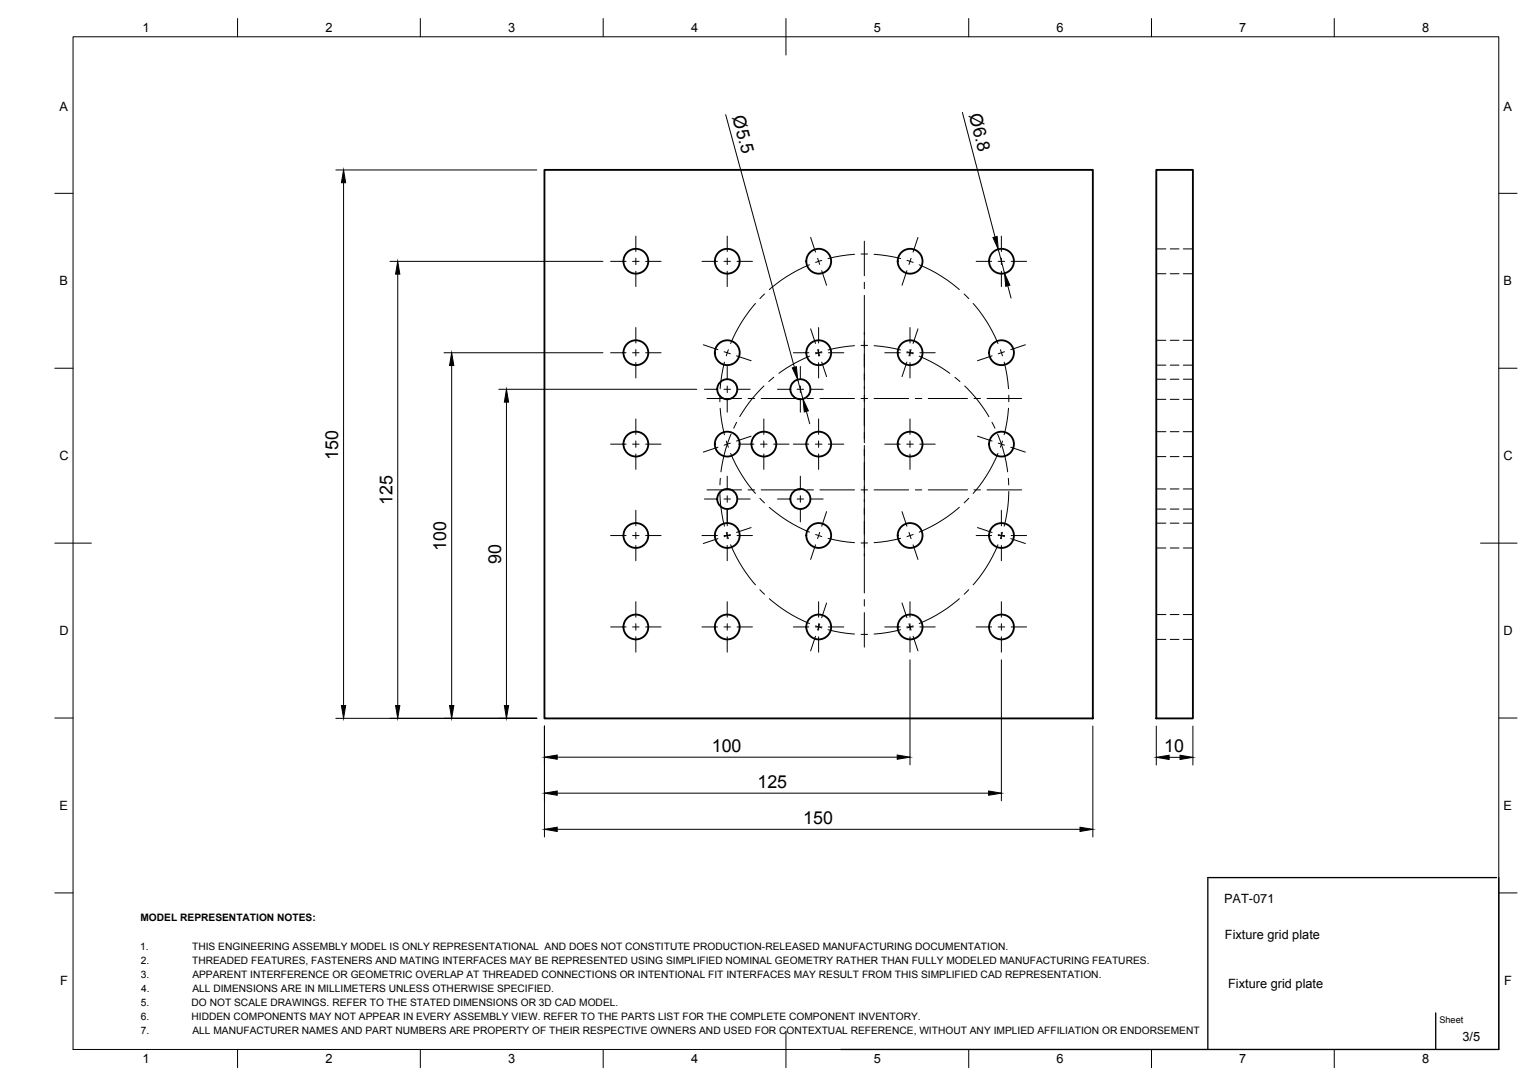
ISO-10303-21;
HEADER;
/* Generated by software containing ST-Developer
 * from STEP Tools, Inc. (www.steptools.com) 
 */

FILE_DESCRIPTION(
/* description */ ('Low-profile wedge edge clamp'),
/* implementation_level */ '2;1');

FILE_NAME(
/* name */ 'Fixture grid plate.step',
/* time_stamp */ '2026-10-29T15:58:13-07:00',
/* author */ (''),
/* organization */ (''),
/* preprocessor_version */ 'ST-DEVELOPER v20.2',
/* originating_system */ 'Autodesk Translation Framework v15.17.0.0',
/* authorisation */ '');

FILE_SCHEMA (('AUTOMOTIVE_DESIGN { 1 0 10303 214 3 1 1 }'));
ENDSEC;

DATA;
#10=MECHANICAL_DESIGN_GEOMETRIC_PRESENTATION_REPRESENTATION('',(#79),#2996);
#67=SHAPE_REPRESENTATION_RELATIONSHIP('SRR','None',#3029,#73);
#73=ADVANCED_BREP_SHAPE_REPRESENTATION('',(#85),#2990);
#79=STYLED_ITEM('',(#3140),#85);
#85=MANIFOLD_SOLID_BREP('Body1',#1708);
#90=FACE_BOUND('',#336,.T.);
#91=FACE_BOUND('',#337,.T.);
#92=FACE_BOUND('',#338,.T.);
#93=FACE_BOUND('',#339,.T.);
#94=FACE_BOUND('',#340,.T.);
#95=FACE_BOUND('',#341,.T.);
#96=FACE_BOUND('',#342,.T.);
#97=FACE_BOUND('',#343,.T.);
#98=FACE_BOUND('',#344,.T.);
#99=FACE_BOUND('',#345,.T.);
#100=FACE_BOUND('',#346,.T.);
#101=FACE_BOUND('',#347,.T.);
#102=FACE_BOUND('',#348,.T.);
#103=FACE_BOUND('',#349,.T.);
#104=FACE_BOUND('',#350,.T.);
#105=FACE_BOUND('',#351,.T.);
#106=FACE_BOUND('',#352,.T.);
#107=FACE_BOUND('',#353,.T.);
#108=FACE_BOUND('',#354,.T.);
#109=FACE_BOUND('',#355,.T.);
#110=FACE_BOUND('',#356,.T.);
#111=FACE_BOUND('',#357,.T.);
#112=FACE_BOUND('',#358,.T.);
#113=FACE_BOUND('',#359,.T.);
#114=FACE_BOUND('',#360,.T.);
#115=FACE_BOUND('',#361,.T.);
#116=FACE_BOUND('',#362,.T.);
#117=FACE_BOUND('',#363,.T.);
#118=FACE_BOUND('',#364,.T.);
#119=FACE_BOUND('',#365,.T.);
#120=FACE_BOUND('',#367,.T.);
#121=FACE_BOUND('',#368,.T.);
#122=FACE_BOUND('',#369,.T.);
#123=FACE_BOUND('',#370,.T.);
#124=FACE_BOUND('',#371,.T.);
#125=FACE_BOUND('',#372,.T.);
#126=FACE_BOUND('',#373,.T.);
#127=FACE_BOUND('',#374,.T.);
#128=FACE_BOUND('',#375,.T.);
#129=FACE_BOUND('',#376,.T.);
#130=FACE_BOUND('',#377,.T.);
#131=FACE_BOUND('',#378,.T.);
#132=FACE_BOUND('',#379,.T.);
#133=FACE_BOUND('',#380,.T.);
#134=FACE_BOUND('',#381,.T.);
#135=FACE_BOUND('',#382,.T.);
#136=FACE_BOUND('',#383,.T.);
#137=FACE_BOUND('',#384,.T.);
#138=FACE_BOUND('',#385,.T.);
#139=FACE_BOUND('',#386,.T.);
#140=FACE_BOUND('',#387,.T.);
#141=FACE_BOUND('',#388,.T.);
#142=FACE_BOUND('',#389,.T.);
#143=FACE_BOUND('',#390,.T.);
#144=FACE_BOUND('',#391,.T.);
#145=FACE_BOUND('',#392,.T.);
#146=FACE_BOUND('',#393,.T.);
#147=FACE_BOUND('',#394,.T.);
#148=FACE_BOUND('',#395,.T.);
#149=FACE_BOUND('',#396,.T.);
#162=PLANE('',#1875);
#163=PLANE('',#1876);
#164=PLANE('',#1877);
#165=PLANE('',#1878);
#166=PLANE('',#1879);
#167=PLANE('',#1880);
#208=FACE_OUTER_BOUND('',#301,.T.);
#209=FACE_OUTER_BOUND('',#302,.T.);
#210=FACE_OUTER_BOUND('',#303,.T.);
#211=FACE_OUTER_BOUND('',#304,.T.);
#212=FACE_OUTER_BOUND('',#305,.T.);
#213=FACE_OUTER_BOUND('',#306,.T.);
#214=FACE_OUTER_BOUND('',#307,.T.);
#215=FACE_OUTER_BOUND('',#308,.T.);
#216=FACE_OUTER_BOUND('',#309,.T.);
#217=FACE_OUTER_BOUND('',#310,.T.);
#218=FACE_OUTER_BOUND('',#311,.T.);
#219=FACE_OUTER_BOUND('',#312,.T.);
#220=FACE_OUTER_BOUND('',#313,.T.);
#221=FACE_OUTER_BOUND('',#314,.T.);
#222=FACE_OUTER_BOUND('',#315,.T.);
#223=FACE_OUTER_BOUND('',#316,.T.);
#224=FACE_OUTER_BOUND('',#317,.T.);
#225=FACE_OUTER_BOUND('',#318,.T.);
#226=FACE_OUTER_BOUND('',#319,.T.);
#227=FACE_OUTER_BOUND('',#320,.T.);
#228=FACE_OUTER_BOUND('',#321,.T.);
#229=FACE_OUTER_BOUND('',#322,.T.);
#230=FACE_OUTER_BOUND('',#323,.T.);
#231=FACE_OUTER_BOUND('',#324,.T.);
#232=FACE_OUTER_BOUND('',#325,.T.);
#233=FACE_OUTER_BOUND('',#326,.T.);
#234=FACE_OUTER_BOUND('',#327,.T.);
#235=FACE_OUTER_BOUND('',#328,.T.);
#236=FACE_OUTER_BOUND('',#329,.T.);
#237=FACE_OUTER_BOUND('',#330,.T.);
#238=FACE_OUTER_BOUND('',#331,.T.);
#239=FACE_OUTER_BOUND('',#332,.T.);
#240=FACE_OUTER_BOUND('',#333,.T.);
#241=FACE_OUTER_BOUND('',#334,.T.);
#242=FACE_OUTER_BOUND('',#335,.T.);
#243=FACE_OUTER_BOUND('',#366,.T.);
#301=EDGE_LOOP('',(#1145,#1146,#1147,#1148));
#302=EDGE_LOOP('',(#1149,#1150,#1151,#1152));
#303=EDGE_LOOP('',(#1153,#1154,#1155,#1156));
#304=EDGE_LOOP('',(#1157,#1158,#1159,#1160));
#305=EDGE_LOOP('',(#1161,#1162,#1163,#1164));
#306=EDGE_LOOP('',(#1165,#1166,#1167,#1168));
#307=EDGE_LOOP('',(#1169,#1170,#1171,#1172));
#308=EDGE_LOOP('',(#1173,#1174,#1175,#1176));
#309=EDGE_LOOP('',(#1177,#1178,#1179,#1180));
#310=EDGE_LOOP('',(#1181,#1182,#1183,#1184));
#311=EDGE_LOOP('',(#1185,#1186,#1187,#1188));
#312=EDGE_LOOP('',(#1189,#1190,#1191,#1192));
#313=EDGE_LOOP('',(#1193,#1194,#1195,#1196));
#314=EDGE_LOOP('',(#1197,#1198,#1199,#1200));
#315=EDGE_LOOP('',(#1201,#1202,#1203,#1204));
#316=EDGE_LOOP('',(#1205,#1206,#1207,#1208));
#317=EDGE_LOOP('',(#1209,#1210,#1211,#1212));
#318=EDGE_LOOP('',(#1213,#1214,#1215,#1216));
#319=EDGE_LOOP('',(#1217,#1218,#1219,#1220));
#320=EDGE_LOOP('',(#1221,#1222,#1223,#1224));
#321=EDGE_LOOP('',(#1225,#1226,#1227,#1228));
#322=EDGE_LOOP('',(#1229,#1230,#1231,#1232));
#323=EDGE_LOOP('',(#1233,#1234,#1235,#1236));
#324=EDGE_LOOP('',(#1237,#1238,#1239,#1240));
#325=EDGE_LOOP('',(#1241,#1242,#1243,#1244));
#326=EDGE_LOOP('',(#1245,#1246,#1247,#1248));
#327=EDGE_LOOP('',(#1249,#1250,#1251,#1252));
#328=EDGE_LOOP('',(#1253,#1254,#1255,#1256));
#329=EDGE_LOOP('',(#1257,#1258,#1259,#1260));
#330=EDGE_LOOP('',(#1261,#1262,#1263,#1264));
#331=EDGE_LOOP('',(#1265,#1266,#1267,#1268));
#332=EDGE_LOOP('',(#1269,#1270,#1271,#1272));
#333=EDGE_LOOP('',(#1273,#1274,#1275,#1276));
#334=EDGE_LOOP('',(#1277,#1278,#1279,#1280));
#335=EDGE_LOOP('',(#1281,#1282,#1283,#1284));
#336=EDGE_LOOP('',(#1285));
#337=EDGE_LOOP('',(#1286));
#338=EDGE_LOOP('',(#1287));
#339=EDGE_LOOP('',(#1288));
#340=EDGE_LOOP('',(#1289));
#341=EDGE_LOOP('',(#1290));
#342=EDGE_LOOP('',(#1291));
#343=EDGE_LOOP('',(#1292));
#344=EDGE_LOOP('',(#1293));
#345=EDGE_LOOP('',(#1294));
#346=EDGE_LOOP('',(#1295));
#347=EDGE_LOOP('',(#1296));
#348=EDGE_LOOP('',(#1297));
#349=EDGE_LOOP('',(#1298));
#350=EDGE_LOOP('',(#1299));
#351=EDGE_LOOP('',(#1300));
#352=EDGE_LOOP('',(#1301));
#353=EDGE_LOOP('',(#1302));
#354=EDGE_LOOP('',(#1303));
#355=EDGE_LOOP('',(#1304));
#356=EDGE_LOOP('',(#1305));
#357=EDGE_LOOP('',(#1306));
#358=EDGE_LOOP('',(#1307));
#359=EDGE_LOOP('',(#1308));
#360=EDGE_LOOP('',(#1309));
#361=EDGE_LOOP('',(#1310));
#362=EDGE_LOOP('',(#1311));
#363=EDGE_LOOP('',(#1312));
#364=EDGE_LOOP('',(#1313));
#365=EDGE_LOOP('',(#1314));
#366=EDGE_LOOP('',(#1315,#1316,#1317,#1318));
#367=EDGE_LOOP('',(#1319));
#368=EDGE_LOOP('',(#1320));
#369=EDGE_LOOP('',(#1321));
#370=EDGE_LOOP('',(#1322));
#371=EDGE_LOOP('',(#1323));
#372=EDGE_LOOP('',(#1324));
#373=EDGE_LOOP('',(#1325));
#374=EDGE_LOOP('',(#1326));
#375=EDGE_LOOP('',(#1327));
#376=EDGE_LOOP('',(#1328));
#377=EDGE_LOOP('',(#1329));
#378=EDGE_LOOP('',(#1330));
#379=EDGE_LOOP('',(#1331));
#380=EDGE_LOOP('',(#1332));
#381=EDGE_LOOP('',(#1333));
#382=EDGE_LOOP('',(#1334));
#383=EDGE_LOOP('',(#1335));
#384=EDGE_LOOP('',(#1336));
#385=EDGE_LOOP('',(#1337));
#386=EDGE_LOOP('',(#1338));
#387=EDGE_LOOP('',(#1339));
#388=EDGE_LOOP('',(#1340));
#389=EDGE_LOOP('',(#1341));
#390=EDGE_LOOP('',(#1342));
#391=EDGE_LOOP('',(#1343));
#392=EDGE_LOOP('',(#1344));
#393=EDGE_LOOP('',(#1345));
#394=EDGE_LOOP('',(#1346));
#395=EDGE_LOOP('',(#1347));
#396=EDGE_LOOP('',(#1348));
#466=LINE('',#2508,#585);
#467=LINE('',#2514,#586);
#468=LINE('',#2520,#587);
#469=LINE('',#2526,#588);
#470=LINE('',#2532,#589);
#471=LINE('',#2538,#590);
#472=LINE('',#2544,#591);
#473=LINE('',#2550,#592);
#474=LINE('',#2556,#593);
#475=LINE('',#2562,#594);
#476=LINE('',#2568,#595);
#477=LINE('',#2574,#596);
#478=LINE('',#2580,#597);
#479=LINE('',#2586,#598);
#480=LINE('',#2592,#599);
#481=LINE('',#2598,#600);
#482=LINE('',#2604,#601);
#483=LINE('',#2610,#602);
#484=LINE('',#2616,#603);
#485=LINE('',#2622,#604);
#486=LINE('',#2628,#605);
#487=LINE('',#2634,#606);
#488=LINE('',#2640,#607);
#489=LINE('',#2646,#608);
#490=LINE('',#2652,#609);
#491=LINE('',#2658,#610);
#492=LINE('',#2664,#611);
#493=LINE('',#2670,#612);
#494=LINE('',#2676,#613);
#495=LINE('',#2682,#614);
#496=LINE('',#2687,#615);
#497=LINE('',#2689,#616);
#498=LINE('',#2691,#617);
#499=LINE('',#2692,#618);
#500=LINE('',#2695,#619);
#501=LINE('',#2697,#620);
#502=LINE('',#2698,#621);
#503=LINE('',#2701,#622);
#504=LINE('',#2703,#623);
#505=LINE('',#2704,#624);
#506=LINE('',#2706,#625);
#507=LINE('',#2707,#626);
#585=VECTOR('',#1992,0.275);
#586=VECTOR('',#1999,0.275);
#587=VECTOR('',#2006,0.275);
#588=VECTOR('',#2013,0.275);
#589=VECTOR('',#2020,0.34);
#590=VECTOR('',#2027,0.34);
#591=VECTOR('',#2034,0.34);
#592=VECTOR('',#2041,0.34);
#593=VECTOR('',#2048,0.34);
#594=VECTOR('',#2055,0.34);
#595=VECTOR('',#2062,0.34);
#596=VECTOR('',#2069,0.34);
#597=VECTOR('',#2076,0.34);
#598=VECTOR('',#2083,0.34);
#599=VECTOR('',#2090,0.34);
#600=VECTOR('',#2097,0.34);
#601=VECTOR('',#2104,0.34);
#602=VECTOR('',#2111,0.34);
#603=VECTOR('',#2118,0.34);
#604=VECTOR('',#2125,0.34);
#605=VECTOR('',#2132,0.34);
#606=VECTOR('',#2139,0.34);
#607=VECTOR('',#2146,0.34);
#608=VECTOR('',#2153,0.34);
#609=VECTOR('',#2160,0.34);
#610=VECTOR('',#2167,0.34);
#611=VECTOR('',#2174,0.34);
#612=VECTOR('',#2181,0.34);
#613=VECTOR('',#2188,0.34);
#614=VECTOR('',#2195,0.34);
#615=VECTOR('',#2200,1.);
#616=VECTOR('',#2201,1.);
#617=VECTOR('',#2202,1.);
#618=VECTOR('',#2203,1.);
#619=VECTOR('',#2206,1.);
#620=VECTOR('',#2207,1.);
#621=VECTOR('',#2208,1.);
#622=VECTOR('',#2211,1.);
#623=VECTOR('',#2212,1.);
#624=VECTOR('',#2213,1.);
#625=VECTOR('',#2216,1.);
#626=VECTOR('',#2217,1.);
#704=CIRCLE('',#1786,0.275);
#705=CIRCLE('',#1787,0.275);
#706=CIRCLE('',#1789,0.275);
#707=CIRCLE('',#1790,0.275);
#708=CIRCLE('',#1792,0.275);
#709=CIRCLE('',#1793,0.275);
#710=CIRCLE('',#1795,0.275);
#711=CIRCLE('',#1796,0.275);
#712=CIRCLE('',#1798,0.34);
#713=CIRCLE('',#1799,0.34);
#714=CIRCLE('',#1801,0.34);
#715=CIRCLE('',#1802,0.34);
#716=CIRCLE('',#1804,0.34);
#717=CIRCLE('',#1805,0.34);
#718=CIRCLE('',#1807,0.34);
#719=CIRCLE('',#1808,0.34);
#720=CIRCLE('',#1810,0.34);
#721=CIRCLE('',#1811,0.34);
#722=CIRCLE('',#1813,0.34);
#723=CIRCLE('',#1814,0.34);
#724=CIRCLE('',#1816,0.34);
#725=CIRCLE('',#1817,0.34);
#726=CIRCLE('',#1819,0.34);
#727=CIRCLE('',#1820,0.34);
#728=CIRCLE('',#1822,0.34);
#729=CIRCLE('',#1823,0.34);
#730=CIRCLE('',#1825,0.34);
#731=CIRCLE('',#1826,0.34);
#732=CIRCLE('',#1828,0.34);
#733=CIRCLE('',#1829,0.34);
#734=CIRCLE('',#1831,0.34);
#735=CIRCLE('',#1832,0.34);
#736=CIRCLE('',#1834,0.34);
#737=CIRCLE('',#1835,0.34);
#738=CIRCLE('',#1837,0.34);
#739=CIRCLE('',#1838,0.34);
#740=CIRCLE('',#1840,0.34);
#741=CIRCLE('',#1841,0.34);
#742=CIRCLE('',#1843,0.34);
#743=CIRCLE('',#1844,0.34);
#744=CIRCLE('',#1846,0.34);
#745=CIRCLE('',#1847,0.34);
#746=CIRCLE('',#1849,0.34);
#747=CIRCLE('',#1850,0.34);
#748=CIRCLE('',#1852,0.34);
#749=CIRCLE('',#1853,0.34);
#750=CIRCLE('',#1855,0.34);
#751=CIRCLE('',#1856,0.34);
#752=CIRCLE('',#1858,0.34);
#753=CIRCLE('',#1859,0.34);
#754=CIRCLE('',#1861,0.34);
#755=CIRCLE('',#1862,0.34);
#756=CIRCLE('',#1864,0.34);
#757=CIRCLE('',#1865,0.34);
#758=CIRCLE('',#1867,0.34);
#759=CIRCLE('',#1868,0.34);
#760=CIRCLE('',#1870,0.34);
#761=CIRCLE('',#1871,0.34);
#762=CIRCLE('',#1873,0.34);
#763=CIRCLE('',#1874,0.34);
#790=VERTEX_POINT('',#2505);
#791=VERTEX_POINT('',#2507);
#792=VERTEX_POINT('',#2511);
#793=VERTEX_POINT('',#2513);
#794=VERTEX_POINT('',#2517);
#795=VERTEX_POINT('',#2519);
#796=VERTEX_POINT('',#2523);
#797=VERTEX_POINT('',#2525);
#798=VERTEX_POINT('',#2529);
#799=VERTEX_POINT('',#2531);
#800=VERTEX_POINT('',#2535);
#801=VERTEX_POINT('',#2537);
#802=VERTEX_POINT('',#2541);
#803=VERTEX_POINT('',#2543);
#804=VERTEX_POINT('',#2547);
#805=VERTEX_POINT('',#2549);
#806=VERTEX_POINT('',#2553);
#807=VERTEX_POINT('',#2555);
#808=VERTEX_POINT('',#2559);
#809=VERTEX_POINT('',#2561);
#810=VERTEX_POINT('',#2565);
#811=VERTEX_POINT('',#2567);
#812=VERTEX_POINT('',#2571);
#813=VERTEX_POINT('',#2573);
#814=VERTEX_POINT('',#2577);
#815=VERTEX_POINT('',#2579);
#816=VERTEX_POINT('',#2583);
#817=VERTEX_POINT('',#2585);
#818=VERTEX_POINT('',#2589);
#819=VERTEX_POINT('',#2591);
#820=VERTEX_POINT('',#2595);
#821=VERTEX_POINT('',#2597);
#822=VERTEX_POINT('',#2601);
#823=VERTEX_POINT('',#2603);
#824=VERTEX_POINT('',#2607);
#825=VERTEX_POINT('',#2609);
#826=VERTEX_POINT('',#2613);
#827=VERTEX_POINT('',#2615);
#828=VERTEX_POINT('',#2619);
#829=VERTEX_POINT('',#2621);
#830=VERTEX_POINT('',#2625);
#831=VERTEX_POINT('',#2627);
#832=VERTEX_POINT('',#2631);
#833=VERTEX_POINT('',#2633);
#834=VERTEX_POINT('',#2637);
#835=VERTEX_POINT('',#2639);
#836=VERTEX_POINT('',#2643);
#837=VERTEX_POINT('',#2645);
#838=VERTEX_POINT('',#2649);
#839=VERTEX_POINT('',#2651);
#840=VERTEX_POINT('',#2655);
#841=VERTEX_POINT('',#2657);
#842=VERTEX_POINT('',#2661);
#843=VERTEX_POINT('',#2663);
#844=VERTEX_POINT('',#2667);
#845=VERTEX_POINT('',#2669);
#846=VERTEX_POINT('',#2673);
#847=VERTEX_POINT('',#2675);
#848=VERTEX_POINT('',#2679);
#849=VERTEX_POINT('',#2681);
#850=VERTEX_POINT('',#2685);
#851=VERTEX_POINT('',#2686);
#852=VERTEX_POINT('',#2688);
#853=VERTEX_POINT('',#2690);
#854=VERTEX_POINT('',#2694);
#855=VERTEX_POINT('',#2696);
#856=VERTEX_POINT('',#2700);
#857=VERTEX_POINT('',#2702);
#931=EDGE_CURVE('',#790,#790,#704,.T.);
#932=EDGE_CURVE('',#790,#791,#466,.T.);
#933=EDGE_CURVE('',#791,#791,#705,.T.);
#934=EDGE_CURVE('',#792,#792,#706,.T.);
#935=EDGE_CURVE('',#792,#793,#467,.T.);
#936=EDGE_CURVE('',#793,#793,#707,.T.);
#937=EDGE_CURVE('',#794,#794,#708,.T.);
#938=EDGE_CURVE('',#794,#795,#468,.T.);
#939=EDGE_CURVE('',#795,#795,#709,.T.);
#940=EDGE_CURVE('',#796,#796,#710,.T.);
#941=EDGE_CURVE('',#796,#797,#469,.T.);
#942=EDGE_CURVE('',#797,#797,#711,.T.);
#943=EDGE_CURVE('',#798,#798,#712,.T.);
#944=EDGE_CURVE('',#798,#799,#470,.T.);
#945=EDGE_CURVE('',#799,#799,#713,.T.);
#946=EDGE_CURVE('',#800,#800,#714,.T.);
#947=EDGE_CURVE('',#800,#801,#471,.T.);
#948=EDGE_CURVE('',#801,#801,#715,.T.);
#949=EDGE_CURVE('',#802,#802,#716,.T.);
#950=EDGE_CURVE('',#802,#803,#472,.T.);
#951=EDGE_CURVE('',#803,#803,#717,.T.);
#952=EDGE_CURVE('',#804,#804,#718,.T.);
#953=EDGE_CURVE('',#804,#805,#473,.T.);
#954=EDGE_CURVE('',#805,#805,#719,.T.);
#955=EDGE_CURVE('',#806,#806,#720,.T.);
#956=EDGE_CURVE('',#806,#807,#474,.T.);
#957=EDGE_CURVE('',#807,#807,#721,.T.);
#958=EDGE_CURVE('',#808,#808,#722,.T.);
#959=EDGE_CURVE('',#808,#809,#475,.T.);
#960=EDGE_CURVE('',#809,#809,#723,.T.);
#961=EDGE_CURVE('',#810,#810,#724,.T.);
#962=EDGE_CURVE('',#810,#811,#476,.T.);
#963=EDGE_CURVE('',#811,#811,#725,.T.);
#964=EDGE_CURVE('',#812,#812,#726,.T.);
#965=EDGE_CURVE('',#812,#813,#477,.T.);
#966=EDGE_CURVE('',#813,#813,#727,.T.);
#967=EDGE_CURVE('',#814,#814,#728,.T.);
#968=EDGE_CURVE('',#814,#815,#478,.T.);
#969=EDGE_CURVE('',#815,#815,#729,.T.);
#970=EDGE_CURVE('',#816,#816,#730,.T.);
#971=EDGE_CURVE('',#816,#817,#479,.T.);
#972=EDGE_CURVE('',#817,#817,#731,.T.);
#973=EDGE_CURVE('',#818,#818,#732,.T.);
#974=EDGE_CURVE('',#818,#819,#480,.T.);
#975=EDGE_CURVE('',#819,#819,#733,.T.);
#976=EDGE_CURVE('',#820,#820,#734,.T.);
#977=EDGE_CURVE('',#820,#821,#481,.T.);
#978=EDGE_CURVE('',#821,#821,#735,.T.);
#979=EDGE_CURVE('',#822,#822,#736,.T.);
#980=EDGE_CURVE('',#822,#823,#482,.T.);
#981=EDGE_CURVE('',#823,#823,#737,.T.);
#982=EDGE_CURVE('',#824,#824,#738,.T.);
#983=EDGE_CURVE('',#824,#825,#483,.T.);
#984=EDGE_CURVE('',#825,#825,#739,.T.);
#985=EDGE_CURVE('',#826,#826,#740,.T.);
#986=EDGE_CURVE('',#826,#827,#484,.T.);
#987=EDGE_CURVE('',#827,#827,#741,.T.);
#988=EDGE_CURVE('',#828,#828,#742,.T.);
#989=EDGE_CURVE('',#828,#829,#485,.T.);
#990=EDGE_CURVE('',#829,#829,#743,.T.);
#991=EDGE_CURVE('',#830,#830,#744,.T.);
#992=EDGE_CURVE('',#830,#831,#486,.T.);
#993=EDGE_CURVE('',#831,#831,#745,.T.);
#994=EDGE_CURVE('',#832,#832,#746,.T.);
#995=EDGE_CURVE('',#832,#833,#487,.T.);
#996=EDGE_CURVE('',#833,#833,#747,.T.);
#997=EDGE_CURVE('',#834,#834,#748,.T.);
#998=EDGE_CURVE('',#834,#835,#488,.T.);
#999=EDGE_CURVE('',#835,#835,#749,.T.);
#1000=EDGE_CURVE('',#836,#836,#750,.T.);
#1001=EDGE_CURVE('',#836,#837,#489,.T.);
#1002=EDGE_CURVE('',#837,#837,#751,.T.);
#1003=EDGE_CURVE('',#838,#838,#752,.T.);
#1004=EDGE_CURVE('',#838,#839,#490,.T.);
#1005=EDGE_CURVE('',#839,#839,#753,.T.);
#1006=EDGE_CURVE('',#840,#840,#754,.T.);
#1007=EDGE_CURVE('',#840,#841,#491,.T.);
#1008=EDGE_CURVE('',#841,#841,#755,.T.);
#1009=EDGE_CURVE('',#842,#842,#756,.T.);
#1010=EDGE_CURVE('',#842,#843,#492,.T.);
#1011=EDGE_CURVE('',#843,#843,#757,.T.);
#1012=EDGE_CURVE('',#844,#844,#758,.T.);
#1013=EDGE_CURVE('',#844,#845,#493,.T.);
#1014=EDGE_CURVE('',#845,#845,#759,.T.);
#1015=EDGE_CURVE('',#846,#846,#760,.T.);
#1016=EDGE_CURVE('',#846,#847,#494,.T.);
#1017=EDGE_CURVE('',#847,#847,#761,.T.);
#1018=EDGE_CURVE('',#848,#848,#762,.T.);
#1019=EDGE_CURVE('',#848,#849,#495,.T.);
#1020=EDGE_CURVE('',#849,#849,#763,.T.);
#1021=EDGE_CURVE('',#850,#851,#496,.T.);
#1022=EDGE_CURVE('',#851,#852,#497,.T.);
#1023=EDGE_CURVE('',#853,#852,#498,.T.);
#1024=EDGE_CURVE('',#850,#853,#499,.T.);
#1025=EDGE_CURVE('',#854,#850,#500,.T.);
#1026=EDGE_CURVE('',#855,#853,#501,.T.);
#1027=EDGE_CURVE('',#854,#855,#502,.T.);
#1028=EDGE_CURVE('',#856,#854,#503,.T.);
#1029=EDGE_CURVE('',#857,#855,#504,.T.);
#1030=EDGE_CURVE('',#856,#857,#505,.T.);
#1031=EDGE_CURVE('',#851,#856,#506,.T.);
#1032=EDGE_CURVE('',#852,#857,#507,.T.);
#1145=ORIENTED_EDGE('',*,*,#931,.F.);
#1146=ORIENTED_EDGE('',*,*,#932,.T.);
#1147=ORIENTED_EDGE('',*,*,#933,.F.);
#1148=ORIENTED_EDGE('',*,*,#932,.F.);
#1149=ORIENTED_EDGE('',*,*,#934,.F.);
#1150=ORIENTED_EDGE('',*,*,#935,.T.);
#1151=ORIENTED_EDGE('',*,*,#936,.F.);
#1152=ORIENTED_EDGE('',*,*,#935,.F.);
#1153=ORIENTED_EDGE('',*,*,#937,.F.);
#1154=ORIENTED_EDGE('',*,*,#938,.T.);
#1155=ORIENTED_EDGE('',*,*,#939,.F.);
#1156=ORIENTED_EDGE('',*,*,#938,.F.);
#1157=ORIENTED_EDGE('',*,*,#940,.F.);
#1158=ORIENTED_EDGE('',*,*,#941,.T.);
#1159=ORIENTED_EDGE('',*,*,#942,.F.);
#1160=ORIENTED_EDGE('',*,*,#941,.F.);
#1161=ORIENTED_EDGE('',*,*,#943,.F.);
#1162=ORIENTED_EDGE('',*,*,#944,.T.);
#1163=ORIENTED_EDGE('',*,*,#945,.F.);
#1164=ORIENTED_EDGE('',*,*,#944,.F.);
#1165=ORIENTED_EDGE('',*,*,#946,.F.);
#1166=ORIENTED_EDGE('',*,*,#947,.T.);
#1167=ORIENTED_EDGE('',*,*,#948,.F.);
#1168=ORIENTED_EDGE('',*,*,#947,.F.);
#1169=ORIENTED_EDGE('',*,*,#949,.F.);
#1170=ORIENTED_EDGE('',*,*,#950,.T.);
#1171=ORIENTED_EDGE('',*,*,#951,.F.);
#1172=ORIENTED_EDGE('',*,*,#950,.F.);
#1173=ORIENTED_EDGE('',*,*,#952,.F.);
#1174=ORIENTED_EDGE('',*,*,#953,.T.);
#1175=ORIENTED_EDGE('',*,*,#954,.F.);
#1176=ORIENTED_EDGE('',*,*,#953,.F.);
#1177=ORIENTED_EDGE('',*,*,#955,.F.);
#1178=ORIENTED_EDGE('',*,*,#956,.T.);
#1179=ORIENTED_EDGE('',*,*,#957,.F.);
#1180=ORIENTED_EDGE('',*,*,#956,.F.);
#1181=ORIENTED_EDGE('',*,*,#958,.F.);
#1182=ORIENTED_EDGE('',*,*,#959,.T.);
#1183=ORIENTED_EDGE('',*,*,#960,.F.);
#1184=ORIENTED_EDGE('',*,*,#959,.F.);
#1185=ORIENTED_EDGE('',*,*,#961,.F.);
#1186=ORIENTED_EDGE('',*,*,#962,.T.);
#1187=ORIENTED_EDGE('',*,*,#963,.F.);
#1188=ORIENTED_EDGE('',*,*,#962,.F.);
#1189=ORIENTED_EDGE('',*,*,#964,.F.);
#1190=ORIENTED_EDGE('',*,*,#965,.T.);
#1191=ORIENTED_EDGE('',*,*,#966,.F.);
#1192=ORIENTED_EDGE('',*,*,#965,.F.);
#1193=ORIENTED_EDGE('',*,*,#967,.F.);
#1194=ORIENTED_EDGE('',*,*,#968,.T.);
#1195=ORIENTED_EDGE('',*,*,#969,.F.);
#1196=ORIENTED_EDGE('',*,*,#968,.F.);
#1197=ORIENTED_EDGE('',*,*,#970,.F.);
#1198=ORIENTED_EDGE('',*,*,#971,.T.);
#1199=ORIENTED_EDGE('',*,*,#972,.F.);
#1200=ORIENTED_EDGE('',*,*,#971,.F.);
#1201=ORIENTED_EDGE('',*,*,#973,.F.);
#1202=ORIENTED_EDGE('',*,*,#974,.T.);
#1203=ORIENTED_EDGE('',*,*,#975,.F.);
#1204=ORIENTED_EDGE('',*,*,#974,.F.);
#1205=ORIENTED_EDGE('',*,*,#976,.F.);
#1206=ORIENTED_EDGE('',*,*,#977,.T.);
#1207=ORIENTED_EDGE('',*,*,#978,.F.);
#1208=ORIENTED_EDGE('',*,*,#977,.F.);
#1209=ORIENTED_EDGE('',*,*,#979,.F.);
#1210=ORIENTED_EDGE('',*,*,#980,.T.);
#1211=ORIENTED_EDGE('',*,*,#981,.F.);
#1212=ORIENTED_EDGE('',*,*,#980,.F.);
#1213=ORIENTED_EDGE('',*,*,#982,.F.);
#1214=ORIENTED_EDGE('',*,*,#983,.T.);
#1215=ORIENTED_EDGE('',*,*,#984,.F.);
#1216=ORIENTED_EDGE('',*,*,#983,.F.);
#1217=ORIENTED_EDGE('',*,*,#985,.F.);
#1218=ORIENTED_EDGE('',*,*,#986,.T.);
#1219=ORIENTED_EDGE('',*,*,#987,.F.);
#1220=ORIENTED_EDGE('',*,*,#986,.F.);
#1221=ORIENTED_EDGE('',*,*,#988,.F.);
#1222=ORIENTED_EDGE('',*,*,#989,.T.);
#1223=ORIENTED_EDGE('',*,*,#990,.F.);
#1224=ORIENTED_EDGE('',*,*,#989,.F.);
#1225=ORIENTED_EDGE('',*,*,#991,.F.);
#1226=ORIENTED_EDGE('',*,*,#992,.T.);
#1227=ORIENTED_EDGE('',*,*,#993,.F.);
#1228=ORIENTED_EDGE('',*,*,#992,.F.);
#1229=ORIENTED_EDGE('',*,*,#994,.F.);
#1230=ORIENTED_EDGE('',*,*,#995,.T.);
#1231=ORIENTED_EDGE('',*,*,#996,.F.);
#1232=ORIENTED_EDGE('',*,*,#995,.F.);
#1233=ORIENTED_EDGE('',*,*,#997,.F.);
#1234=ORIENTED_EDGE('',*,*,#998,.T.);
#1235=ORIENTED_EDGE('',*,*,#999,.F.);
#1236=ORIENTED_EDGE('',*,*,#998,.F.);
#1237=ORIENTED_EDGE('',*,*,#1000,.F.);
#1238=ORIENTED_EDGE('',*,*,#1001,.T.);
#1239=ORIENTED_EDGE('',*,*,#1002,.F.);
#1240=ORIENTED_EDGE('',*,*,#1001,.F.);
#1241=ORIENTED_EDGE('',*,*,#1003,.F.);
#1242=ORIENTED_EDGE('',*,*,#1004,.T.);
#1243=ORIENTED_EDGE('',*,*,#1005,.F.);
#1244=ORIENTED_EDGE('',*,*,#1004,.F.);
#1245=ORIENTED_EDGE('',*,*,#1006,.F.);
#1246=ORIENTED_EDGE('',*,*,#1007,.T.);
#1247=ORIENTED_EDGE('',*,*,#1008,.F.);
#1248=ORIENTED_EDGE('',*,*,#1007,.F.);
#1249=ORIENTED_EDGE('',*,*,#1009,.F.);
#1250=ORIENTED_EDGE('',*,*,#1010,.T.);
#1251=ORIENTED_EDGE('',*,*,#1011,.F.);
#1252=ORIENTED_EDGE('',*,*,#1010,.F.);
#1253=ORIENTED_EDGE('',*,*,#1012,.F.);
#1254=ORIENTED_EDGE('',*,*,#1013,.T.);
#1255=ORIENTED_EDGE('',*,*,#1014,.F.);
#1256=ORIENTED_EDGE('',*,*,#1013,.F.);
#1257=ORIENTED_EDGE('',*,*,#1015,.F.);
#1258=ORIENTED_EDGE('',*,*,#1016,.T.);
#1259=ORIENTED_EDGE('',*,*,#1017,.F.);
#1260=ORIENTED_EDGE('',*,*,#1016,.F.);
#1261=ORIENTED_EDGE('',*,*,#1018,.F.);
#1262=ORIENTED_EDGE('',*,*,#1019,.T.);
#1263=ORIENTED_EDGE('',*,*,#1020,.F.);
#1264=ORIENTED_EDGE('',*,*,#1019,.F.);
#1265=ORIENTED_EDGE('',*,*,#1021,.T.);
#1266=ORIENTED_EDGE('',*,*,#1022,.T.);
#1267=ORIENTED_EDGE('',*,*,#1023,.F.);
#1268=ORIENTED_EDGE('',*,*,#1024,.F.);
#1269=ORIENTED_EDGE('',*,*,#1025,.T.);
#1270=ORIENTED_EDGE('',*,*,#1024,.T.);
#1271=ORIENTED_EDGE('',*,*,#1026,.F.);
#1272=ORIENTED_EDGE('',*,*,#1027,.F.);
#1273=ORIENTED_EDGE('',*,*,#1028,.T.);
#1274=ORIENTED_EDGE('',*,*,#1027,.T.);
#1275=ORIENTED_EDGE('',*,*,#1029,.F.);
#1276=ORIENTED_EDGE('',*,*,#1030,.F.);
#1277=ORIENTED_EDGE('',*,*,#1031,.T.);
#1278=ORIENTED_EDGE('',*,*,#1030,.T.);
#1279=ORIENTED_EDGE('',*,*,#1032,.F.);
#1280=ORIENTED_EDGE('',*,*,#1022,.F.);
#1281=ORIENTED_EDGE('',*,*,#1032,.T.);
#1282=ORIENTED_EDGE('',*,*,#1029,.T.);
#1283=ORIENTED_EDGE('',*,*,#1026,.T.);
#1284=ORIENTED_EDGE('',*,*,#1023,.T.);
#1285=ORIENTED_EDGE('',*,*,#945,.T.);
#1286=ORIENTED_EDGE('',*,*,#1020,.T.);
#1287=ORIENTED_EDGE('',*,*,#1017,.T.);
#1288=ORIENTED_EDGE('',*,*,#1014,.T.);
#1289=ORIENTED_EDGE('',*,*,#1011,.T.);
#1290=ORIENTED_EDGE('',*,*,#1008,.T.);
#1291=ORIENTED_EDGE('',*,*,#1005,.T.);
#1292=ORIENTED_EDGE('',*,*,#1002,.T.);
#1293=ORIENTED_EDGE('',*,*,#999,.T.);
#1294=ORIENTED_EDGE('',*,*,#996,.T.);
#1295=ORIENTED_EDGE('',*,*,#993,.T.);
#1296=ORIENTED_EDGE('',*,*,#990,.T.);
#1297=ORIENTED_EDGE('',*,*,#987,.T.);
#1298=ORIENTED_EDGE('',*,*,#984,.T.);
#1299=ORIENTED_EDGE('',*,*,#981,.T.);
#1300=ORIENTED_EDGE('',*,*,#978,.T.);
#1301=ORIENTED_EDGE('',*,*,#975,.T.);
#1302=ORIENTED_EDGE('',*,*,#972,.T.);
#1303=ORIENTED_EDGE('',*,*,#969,.T.);
#1304=ORIENTED_EDGE('',*,*,#966,.T.);
#1305=ORIENTED_EDGE('',*,*,#963,.T.);
#1306=ORIENTED_EDGE('',*,*,#960,.T.);
#1307=ORIENTED_EDGE('',*,*,#957,.T.);
#1308=ORIENTED_EDGE('',*,*,#954,.T.);
#1309=ORIENTED_EDGE('',*,*,#951,.T.);
#1310=ORIENTED_EDGE('',*,*,#948,.T.);
#1311=ORIENTED_EDGE('',*,*,#942,.T.);
#1312=ORIENTED_EDGE('',*,*,#939,.T.);
#1313=ORIENTED_EDGE('',*,*,#936,.T.);
#1314=ORIENTED_EDGE('',*,*,#933,.T.);
#1315=ORIENTED_EDGE('',*,*,#1031,.F.);
#1316=ORIENTED_EDGE('',*,*,#1021,.F.);
#1317=ORIENTED_EDGE('',*,*,#1025,.F.);
#1318=ORIENTED_EDGE('',*,*,#1028,.F.);
#1319=ORIENTED_EDGE('',*,*,#943,.T.);
#1320=ORIENTED_EDGE('',*,*,#1018,.T.);
#1321=ORIENTED_EDGE('',*,*,#1015,.T.);
#1322=ORIENTED_EDGE('',*,*,#1012,.T.);
#1323=ORIENTED_EDGE('',*,*,#1009,.T.);
#1324=ORIENTED_EDGE('',*,*,#1006,.T.);
#1325=ORIENTED_EDGE('',*,*,#1003,.T.);
#1326=ORIENTED_EDGE('',*,*,#1000,.T.);
#1327=ORIENTED_EDGE('',*,*,#997,.T.);
#1328=ORIENTED_EDGE('',*,*,#994,.T.);
#1329=ORIENTED_EDGE('',*,*,#991,.T.);
#1330=ORIENTED_EDGE('',*,*,#988,.T.);
#1331=ORIENTED_EDGE('',*,*,#985,.T.);
#1332=ORIENTED_EDGE('',*,*,#982,.T.);
#1333=ORIENTED_EDGE('',*,*,#979,.T.);
#1334=ORIENTED_EDGE('',*,*,#976,.T.);
#1335=ORIENTED_EDGE('',*,*,#973,.T.);
#1336=ORIENTED_EDGE('',*,*,#970,.T.);
#1337=ORIENTED_EDGE('',*,*,#967,.T.);
#1338=ORIENTED_EDGE('',*,*,#964,.T.);
#1339=ORIENTED_EDGE('',*,*,#961,.T.);
#1340=ORIENTED_EDGE('',*,*,#958,.T.);
#1341=ORIENTED_EDGE('',*,*,#955,.T.);
#1342=ORIENTED_EDGE('',*,*,#952,.T.);
#1343=ORIENTED_EDGE('',*,*,#949,.T.);
#1344=ORIENTED_EDGE('',*,*,#946,.T.);
#1345=ORIENTED_EDGE('',*,*,#940,.T.);
#1346=ORIENTED_EDGE('',*,*,#937,.T.);
#1347=ORIENTED_EDGE('',*,*,#934,.T.);
#1348=ORIENTED_EDGE('',*,*,#931,.T.);
#1573=CYLINDRICAL_SURFACE('',#1785,0.275);
#1574=CYLINDRICAL_SURFACE('',#1788,0.275);
#1575=CYLINDRICAL_SURFACE('',#1791,0.275);
#1576=CYLINDRICAL_SURFACE('',#1794,0.275);
#1577=CYLINDRICAL_SURFACE('',#1797,0.34);
#1578=CYLINDRICAL_SURFACE('',#1800,0.34);
#1579=CYLINDRICAL_SURFACE('',#1803,0.34);
#1580=CYLINDRICAL_SURFACE('',#1806,0.34);
#1581=CYLINDRICAL_SURFACE('',#1809,0.34);
#1582=CYLINDRICAL_SURFACE('',#1812,0.34);
#1583=CYLINDRICAL_SURFACE('',#1815,0.34);
#1584=CYLINDRICAL_SURFACE('',#1818,0.34);
#1585=CYLINDRICAL_SURFACE('',#1821,0.34);
#1586=CYLINDRICAL_SURFACE('',#1824,0.34);
#1587=CYLINDRICAL_SURFACE('',#1827,0.34);
#1588=CYLINDRICAL_SURFACE('',#1830,0.34);
#1589=CYLINDRICAL_SURFACE('',#1833,0.34);
#1590=CYLINDRICAL_SURFACE('',#1836,0.34);
#1591=CYLINDRICAL_SURFACE('',#1839,0.34);
#1592=CYLINDRICAL_SURFACE('',#1842,0.34);
#1593=CYLINDRICAL_SURFACE('',#1845,0.34);
#1594=CYLINDRICAL_SURFACE('',#1848,0.34);
#1595=CYLINDRICAL_SURFACE('',#1851,0.34);
#1596=CYLINDRICAL_SURFACE('',#1854,0.34);
#1597=CYLINDRICAL_SURFACE('',#1857,0.34);
#1598=CYLINDRICAL_SURFACE('',#1860,0.34);
#1599=CYLINDRICAL_SURFACE('',#1863,0.34);
#1600=CYLINDRICAL_SURFACE('',#1866,0.34);
#1601=CYLINDRICAL_SURFACE('',#1869,0.34);
#1602=CYLINDRICAL_SURFACE('',#1872,0.34);
#1615=ADVANCED_FACE('',(#208),#1573,.F.);
#1616=ADVANCED_FACE('',(#209),#1574,.F.);
#1617=ADVANCED_FACE('',(#210),#1575,.F.);
#1618=ADVANCED_FACE('',(#211),#1576,.F.);
#1619=ADVANCED_FACE('',(#212),#1577,.F.);
#1620=ADVANCED_FACE('',(#213),#1578,.F.);
#1621=ADVANCED_FACE('',(#214),#1579,.F.);
#1622=ADVANCED_FACE('',(#215),#1580,.F.);
#1623=ADVANCED_FACE('',(#216),#1581,.F.);
#1624=ADVANCED_FACE('',(#217),#1582,.F.);
#1625=ADVANCED_FACE('',(#218),#1583,.F.);
#1626=ADVANCED_FACE('',(#219),#1584,.F.);
#1627=ADVANCED_FACE('',(#220),#1585,.F.);
#1628=ADVANCED_FACE('',(#221),#1586,.F.);
#1629=ADVANCED_FACE('',(#222),#1587,.F.);
#1630=ADVANCED_FACE('',(#223),#1588,.F.);
#1631=ADVANCED_FACE('',(#224),#1589,.F.);
#1632=ADVANCED_FACE('',(#225),#1590,.F.);
#1633=ADVANCED_FACE('',(#226),#1591,.F.);
#1634=ADVANCED_FACE('',(#227),#1592,.F.);
#1635=ADVANCED_FACE('',(#228),#1593,.F.);
#1636=ADVANCED_FACE('',(#229),#1594,.F.);
#1637=ADVANCED_FACE('',(#230),#1595,.F.);
#1638=ADVANCED_FACE('',(#231),#1596,.F.);
#1639=ADVANCED_FACE('',(#232),#1597,.F.);
#1640=ADVANCED_FACE('',(#233),#1598,.F.);
#1641=ADVANCED_FACE('',(#234),#1599,.F.);
#1642=ADVANCED_FACE('',(#235),#1600,.F.);
#1643=ADVANCED_FACE('',(#236),#1601,.F.);
#1644=ADVANCED_FACE('',(#237),#1602,.F.);
#1645=ADVANCED_FACE('',(#238),#162,.T.);
#1646=ADVANCED_FACE('',(#239),#163,.T.);
#1647=ADVANCED_FACE('',(#240),#164,.T.);
#1648=ADVANCED_FACE('',(#241),#165,.T.);
#1649=ADVANCED_FACE('',(#242,#90,#91,#92,#93,#94,#95,#96,#97,#98,#99,#100,
#101,#102,#103,#104,#105,#106,#107,#108,#109,#110,#111,#112,#113,#114,#115,
#116,#117,#118,#119),#166,.T.);
#1650=ADVANCED_FACE('',(#243,#120,#121,#122,#123,#124,#125,#126,#127,#128,
#129,#130,#131,#132,#133,#134,#135,#136,#137,#138,#139,#140,#141,#142,#143,
#144,#145,#146,#147,#148,#149),#167,.F.);
#1708=CLOSED_SHELL('',(#1615,#1616,#1617,#1618,#1619,#1620,#1621,#1622,
#1623,#1624,#1625,#1626,#1627,#1628,#1629,#1630,#1631,#1632,#1633,#1634,
#1635,#1636,#1637,#1638,#1639,#1640,#1641,#1642,#1643,#1644,#1645,#1646,
#1647,#1648,#1649,#1650));
#1784=AXIS2_PLACEMENT_3D('',#2503,#1986,#1987);
#1785=AXIS2_PLACEMENT_3D('',#2504,#1988,#1989);
#1786=AXIS2_PLACEMENT_3D('',#2506,#1990,#1991);
#1787=AXIS2_PLACEMENT_3D('',#2509,#1993,#1994);
#1788=AXIS2_PLACEMENT_3D('',#2510,#1995,#1996);
#1789=AXIS2_PLACEMENT_3D('',#2512,#1997,#1998);
#1790=AXIS2_PLACEMENT_3D('',#2515,#2000,#2001);
#1791=AXIS2_PLACEMENT_3D('',#2516,#2002,#2003);
#1792=AXIS2_PLACEMENT_3D('',#2518,#2004,#2005);
#1793=AXIS2_PLACEMENT_3D('',#2521,#2007,#2008);
#1794=AXIS2_PLACEMENT_3D('',#2522,#2009,#2010);
#1795=AXIS2_PLACEMENT_3D('',#2524,#2011,#2012);
#1796=AXIS2_PLACEMENT_3D('',#2527,#2014,#2015);
#1797=AXIS2_PLACEMENT_3D('',#2528,#2016,#2017);
#1798=AXIS2_PLACEMENT_3D('',#2530,#2018,#2019);
#1799=AXIS2_PLACEMENT_3D('',#2533,#2021,#2022);
#1800=AXIS2_PLACEMENT_3D('',#2534,#2023,#2024);
#1801=AXIS2_PLACEMENT_3D('',#2536,#2025,#2026);
#1802=AXIS2_PLACEMENT_3D('',#2539,#2028,#2029);
#1803=AXIS2_PLACEMENT_3D('',#2540,#2030,#2031);
#1804=AXIS2_PLACEMENT_3D('',#2542,#2032,#2033);
#1805=AXIS2_PLACEMENT_3D('',#2545,#2035,#2036);
#1806=AXIS2_PLACEMENT_3D('',#2546,#2037,#2038);
#1807=AXIS2_PLACEMENT_3D('',#2548,#2039,#2040);
#1808=AXIS2_PLACEMENT_3D('',#2551,#2042,#2043);
#1809=AXIS2_PLACEMENT_3D('',#2552,#2044,#2045);
#1810=AXIS2_PLACEMENT_3D('',#2554,#2046,#2047);
#1811=AXIS2_PLACEMENT_3D('',#2557,#2049,#2050);
#1812=AXIS2_PLACEMENT_3D('',#2558,#2051,#2052);
#1813=AXIS2_PLACEMENT_3D('',#2560,#2053,#2054);
#1814=AXIS2_PLACEMENT_3D('',#2563,#2056,#2057);
#1815=AXIS2_PLACEMENT_3D('',#2564,#2058,#2059);
#1816=AXIS2_PLACEMENT_3D('',#2566,#2060,#2061);
#1817=AXIS2_PLACEMENT_3D('',#2569,#2063,#2064);
#1818=AXIS2_PLACEMENT_3D('',#2570,#2065,#2066);
#1819=AXIS2_PLACEMENT_3D('',#2572,#2067,#2068);
#1820=AXIS2_PLACEMENT_3D('',#2575,#2070,#2071);
#1821=AXIS2_PLACEMENT_3D('',#2576,#2072,#2073);
#1822=AXIS2_PLACEMENT_3D('',#2578,#2074,#2075);
#1823=AXIS2_PLACEMENT_3D('',#2581,#2077,#2078);
#1824=AXIS2_PLACEMENT_3D('',#2582,#2079,#2080);
#1825=AXIS2_PLACEMENT_3D('',#2584,#2081,#2082);
#1826=AXIS2_PLACEMENT_3D('',#2587,#2084,#2085);
#1827=AXIS2_PLACEMENT_3D('',#2588,#2086,#2087);
#1828=AXIS2_PLACEMENT_3D('',#2590,#2088,#2089);
#1829=AXIS2_PLACEMENT_3D('',#2593,#2091,#2092);
#1830=AXIS2_PLACEMENT_3D('',#2594,#2093,#2094);
#1831=AXIS2_PLACEMENT_3D('',#2596,#2095,#2096);
#1832=AXIS2_PLACEMENT_3D('',#2599,#2098,#2099);
#1833=AXIS2_PLACEMENT_3D('',#2600,#2100,#2101);
#1834=AXIS2_PLACEMENT_3D('',#2602,#2102,#2103);
#1835=AXIS2_PLACEMENT_3D('',#2605,#2105,#2106);
#1836=AXIS2_PLACEMENT_3D('',#2606,#2107,#2108);
#1837=AXIS2_PLACEMENT_3D('',#2608,#2109,#2110);
#1838=AXIS2_PLACEMENT_3D('',#2611,#2112,#2113);
#1839=AXIS2_PLACEMENT_3D('',#2612,#2114,#2115);
#1840=AXIS2_PLACEMENT_3D('',#2614,#2116,#2117);
#1841=AXIS2_PLACEMENT_3D('',#2617,#2119,#2120);
#1842=AXIS2_PLACEMENT_3D('',#2618,#2121,#2122);
#1843=AXIS2_PLACEMENT_3D('',#2620,#2123,#2124);
#1844=AXIS2_PLACEMENT_3D('',#2623,#2126,#2127);
#1845=AXIS2_PLACEMENT_3D('',#2624,#2128,#2129);
#1846=AXIS2_PLACEMENT_3D('',#2626,#2130,#2131);
#1847=AXIS2_PLACEMENT_3D('',#2629,#2133,#2134);
#1848=AXIS2_PLACEMENT_3D('',#2630,#2135,#2136);
#1849=AXIS2_PLACEMENT_3D('',#2632,#2137,#2138);
#1850=AXIS2_PLACEMENT_3D('',#2635,#2140,#2141);
#1851=AXIS2_PLACEMENT_3D('',#2636,#2142,#2143);
#1852=AXIS2_PLACEMENT_3D('',#2638,#2144,#2145);
#1853=AXIS2_PLACEMENT_3D('',#2641,#2147,#2148);
#1854=AXIS2_PLACEMENT_3D('',#2642,#2149,#2150);
#1855=AXIS2_PLACEMENT_3D('',#2644,#2151,#2152);
#1856=AXIS2_PLACEMENT_3D('',#2647,#2154,#2155);
#1857=AXIS2_PLACEMENT_3D('',#2648,#2156,#2157);
#1858=AXIS2_PLACEMENT_3D('',#2650,#2158,#2159);
#1859=AXIS2_PLACEMENT_3D('',#2653,#2161,#2162);
#1860=AXIS2_PLACEMENT_3D('',#2654,#2163,#2164);
#1861=AXIS2_PLACEMENT_3D('',#2656,#2165,#2166);
#1862=AXIS2_PLACEMENT_3D('',#2659,#2168,#2169);
#1863=AXIS2_PLACEMENT_3D('',#2660,#2170,#2171);
#1864=AXIS2_PLACEMENT_3D('',#2662,#2172,#2173);
#1865=AXIS2_PLACEMENT_3D('',#2665,#2175,#2176);
#1866=AXIS2_PLACEMENT_3D('',#2666,#2177,#2178);
#1867=AXIS2_PLACEMENT_3D('',#2668,#2179,#2180);
#1868=AXIS2_PLACEMENT_3D('',#2671,#2182,#2183);
#1869=AXIS2_PLACEMENT_3D('',#2672,#2184,#2185);
#1870=AXIS2_PLACEMENT_3D('',#2674,#2186,#2187);
#1871=AXIS2_PLACEMENT_3D('',#2677,#2189,#2190);
#1872=AXIS2_PLACEMENT_3D('',#2678,#2191,#2192);
#1873=AXIS2_PLACEMENT_3D('',#2680,#2193,#2194);
#1874=AXIS2_PLACEMENT_3D('',#2683,#2196,#2197);
#1875=AXIS2_PLACEMENT_3D('',#2684,#2198,#2199);
#1876=AXIS2_PLACEMENT_3D('',#2693,#2204,#2205);
#1877=AXIS2_PLACEMENT_3D('',#2699,#2209,#2210);
#1878=AXIS2_PLACEMENT_3D('',#2705,#2214,#2215);
#1879=AXIS2_PLACEMENT_3D('',#2708,#2218,#2219);
#1880=AXIS2_PLACEMENT_3D('',#2709,#2220,#2221);
#1986=DIRECTION('axis',(0.,0.,1.));
#1987=DIRECTION('refdir',(1.,0.,0.));
#1988=DIRECTION('center_axis',(0.,0.,1.));
#1989=DIRECTION('ref_axis',(1.,0.,0.));
#1990=DIRECTION('center_axis',(0.,0.,1.));
#1991=DIRECTION('ref_axis',(1.,0.,0.));
#1992=DIRECTION('',(0.,0.,1.));
#1993=DIRECTION('center_axis',(0.,0.,-1.));
#1994=DIRECTION('ref_axis',(1.,0.,0.));
#1995=DIRECTION('center_axis',(0.,0.,1.));
#1996=DIRECTION('ref_axis',(1.,0.,0.));
#1997=DIRECTION('center_axis',(0.,0.,1.));
#1998=DIRECTION('ref_axis',(1.,0.,0.));
#1999=DIRECTION('',(0.,0.,1.));
#2000=DIRECTION('center_axis',(0.,0.,-1.));
#2001=DIRECTION('ref_axis',(1.,0.,0.));
#2002=DIRECTION('center_axis',(0.,0.,1.));
#2003=DIRECTION('ref_axis',(1.,0.,0.));
#2004=DIRECTION('center_axis',(0.,0.,1.));
#2005=DIRECTION('ref_axis',(1.,0.,0.));
#2006=DIRECTION('',(0.,0.,1.));
#2007=DIRECTION('center_axis',(0.,0.,-1.));
#2008=DIRECTION('ref_axis',(1.,0.,0.));
#2009=DIRECTION('center_axis',(0.,0.,1.));
#2010=DIRECTION('ref_axis',(1.,0.,0.));
#2011=DIRECTION('center_axis',(0.,0.,1.));
#2012=DIRECTION('ref_axis',(1.,0.,0.));
#2013=DIRECTION('',(0.,0.,1.));
#2014=DIRECTION('center_axis',(0.,0.,-1.));
#2015=DIRECTION('ref_axis',(1.,0.,0.));
#2016=DIRECTION('center_axis',(0.,0.,1.));
#2017=DIRECTION('ref_axis',(1.,0.,0.));
#2018=DIRECTION('center_axis',(0.,0.,1.));
#2019=DIRECTION('ref_axis',(1.,0.,0.));
#2020=DIRECTION('',(0.,0.,1.));
#2021=DIRECTION('center_axis',(0.,0.,-1.));
#2022=DIRECTION('ref_axis',(1.,0.,0.));
#2023=DIRECTION('center_axis',(0.,0.,1.));
#2024=DIRECTION('ref_axis',(1.,0.,0.));
#2025=DIRECTION('center_axis',(0.,0.,1.));
#2026=DIRECTION('ref_axis',(1.,0.,0.));
#2027=DIRECTION('',(0.,0.,1.));
#2028=DIRECTION('center_axis',(0.,0.,-1.));
#2029=DIRECTION('ref_axis',(1.,0.,0.));
#2030=DIRECTION('center_axis',(0.,0.,1.));
#2031=DIRECTION('ref_axis',(1.,0.,0.));
#2032=DIRECTION('center_axis',(0.,0.,1.));
#2033=DIRECTION('ref_axis',(1.,0.,0.));
#2034=DIRECTION('',(0.,0.,1.));
#2035=DIRECTION('center_axis',(0.,0.,-1.));
#2036=DIRECTION('ref_axis',(1.,0.,0.));
#2037=DIRECTION('center_axis',(0.,0.,1.));
#2038=DIRECTION('ref_axis',(1.,0.,0.));
#2039=DIRECTION('center_axis',(0.,0.,1.));
#2040=DIRECTION('ref_axis',(1.,0.,0.));
#2041=DIRECTION('',(0.,0.,1.));
#2042=DIRECTION('center_axis',(0.,0.,-1.));
#2043=DIRECTION('ref_axis',(1.,0.,0.));
#2044=DIRECTION('center_axis',(0.,0.,1.));
#2045=DIRECTION('ref_axis',(1.,0.,0.));
#2046=DIRECTION('center_axis',(0.,0.,1.));
#2047=DIRECTION('ref_axis',(1.,0.,0.));
#2048=DIRECTION('',(0.,0.,1.));
#2049=DIRECTION('center_axis',(0.,0.,-1.));
#2050=DIRECTION('ref_axis',(1.,0.,0.));
#2051=DIRECTION('center_axis',(0.,0.,1.));
#2052=DIRECTION('ref_axis',(1.,0.,0.));
#2053=DIRECTION('center_axis',(0.,0.,1.));
#2054=DIRECTION('ref_axis',(1.,0.,0.));
#2055=DIRECTION('',(0.,0.,1.));
#2056=DIRECTION('center_axis',(0.,0.,-1.));
#2057=DIRECTION('ref_axis',(1.,0.,0.));
#2058=DIRECTION('center_axis',(0.,0.,1.));
#2059=DIRECTION('ref_axis',(1.,0.,0.));
#2060=DIRECTION('center_axis',(0.,0.,1.));
#2061=DIRECTION('ref_axis',(1.,0.,0.));
#2062=DIRECTION('',(0.,0.,1.));
#2063=DIRECTION('center_axis',(0.,0.,-1.));
#2064=DIRECTION('ref_axis',(1.,0.,0.));
#2065=DIRECTION('center_axis',(0.,0.,1.));
#2066=DIRECTION('ref_axis',(1.,0.,0.));
#2067=DIRECTION('center_axis',(0.,0.,1.));
#2068=DIRECTION('ref_axis',(1.,0.,0.));
#2069=DIRECTION('',(0.,0.,1.));
#2070=DIRECTION('center_axis',(0.,0.,-1.));
#2071=DIRECTION('ref_axis',(1.,0.,0.));
#2072=DIRECTION('center_axis',(0.,0.,1.));
#2073=DIRECTION('ref_axis',(1.,0.,0.));
#2074=DIRECTION('center_axis',(0.,0.,1.));
#2075=DIRECTION('ref_axis',(1.,0.,0.));
#2076=DIRECTION('',(0.,0.,1.));
#2077=DIRECTION('center_axis',(0.,0.,-1.));
#2078=DIRECTION('ref_axis',(1.,0.,0.));
#2079=DIRECTION('center_axis',(0.,0.,1.));
#2080=DIRECTION('ref_axis',(1.,0.,0.));
#2081=DIRECTION('center_axis',(0.,0.,1.));
#2082=DIRECTION('ref_axis',(1.,0.,0.));
#2083=DIRECTION('',(0.,0.,1.));
#2084=DIRECTION('center_axis',(0.,0.,-1.));
#2085=DIRECTION('ref_axis',(1.,0.,0.));
#2086=DIRECTION('center_axis',(0.,0.,1.));
#2087=DIRECTION('ref_axis',(1.,0.,0.));
#2088=DIRECTION('center_axis',(0.,0.,1.));
#2089=DIRECTION('ref_axis',(1.,0.,0.));
#2090=DIRECTION('',(0.,0.,1.));
#2091=DIRECTION('center_axis',(0.,0.,-1.));
#2092=DIRECTION('ref_axis',(1.,0.,0.));
#2093=DIRECTION('center_axis',(0.,0.,1.));
#2094=DIRECTION('ref_axis',(1.,0.,0.));
#2095=DIRECTION('center_axis',(0.,0.,1.));
#2096=DIRECTION('ref_axis',(1.,0.,0.));
#2097=DIRECTION('',(0.,0.,1.));
#2098=DIRECTION('center_axis',(0.,0.,-1.));
#2099=DIRECTION('ref_axis',(1.,0.,0.));
#2100=DIRECTION('center_axis',(0.,0.,1.));
#2101=DIRECTION('ref_axis',(1.,0.,0.));
#2102=DIRECTION('center_axis',(0.,0.,1.));
#2103=DIRECTION('ref_axis',(1.,0.,0.));
#2104=DIRECTION('',(0.,0.,1.));
#2105=DIRECTION('center_axis',(0.,0.,-1.));
#2106=DIRECTION('ref_axis',(1.,0.,0.));
#2107=DIRECTION('center_axis',(0.,0.,1.));
#2108=DIRECTION('ref_axis',(1.,0.,0.));
#2109=DIRECTION('center_axis',(0.,0.,1.));
#2110=DIRECTION('ref_axis',(1.,0.,0.));
#2111=DIRECTION('',(0.,0.,1.));
#2112=DIRECTION('center_axis',(0.,0.,-1.));
#2113=DIRECTION('ref_axis',(1.,0.,0.));
#2114=DIRECTION('center_axis',(0.,0.,1.));
#2115=DIRECTION('ref_axis',(1.,0.,0.));
#2116=DIRECTION('center_axis',(0.,0.,1.));
#2117=DIRECTION('ref_axis',(1.,0.,0.));
#2118=DIRECTION('',(0.,0.,1.));
#2119=DIRECTION('center_axis',(0.,0.,-1.));
#2120=DIRECTION('ref_axis',(1.,0.,0.));
#2121=DIRECTION('center_axis',(0.,0.,1.));
#2122=DIRECTION('ref_axis',(1.,0.,0.));
#2123=DIRECTION('center_axis',(0.,0.,1.));
#2124=DIRECTION('ref_axis',(1.,0.,0.));
#2125=DIRECTION('',(0.,0.,1.));
#2126=DIRECTION('center_axis',(0.,0.,-1.));
#2127=DIRECTION('ref_axis',(1.,0.,0.));
#2128=DIRECTION('center_axis',(0.,0.,1.));
#2129=DIRECTION('ref_axis',(1.,0.,0.));
#2130=DIRECTION('center_axis',(0.,0.,1.));
#2131=DIRECTION('ref_axis',(1.,0.,0.));
#2132=DIRECTION('',(0.,0.,1.));
#2133=DIRECTION('center_axis',(0.,0.,-1.));
#2134=DIRECTION('ref_axis',(1.,0.,0.));
#2135=DIRECTION('center_axis',(0.,0.,1.));
#2136=DIRECTION('ref_axis',(1.,0.,0.));
#2137=DIRECTION('center_axis',(0.,0.,1.));
#2138=DIRECTION('ref_axis',(1.,0.,0.));
#2139=DIRECTION('',(0.,0.,1.));
#2140=DIRECTION('center_axis',(0.,0.,-1.));
#2141=DIRECTION('ref_axis',(1.,0.,0.));
#2142=DIRECTION('center_axis',(0.,0.,1.));
#2143=DIRECTION('ref_axis',(1.,0.,0.));
#2144=DIRECTION('center_axis',(0.,0.,1.));
#2145=DIRECTION('ref_axis',(1.,0.,0.));
#2146=DIRECTION('',(0.,0.,1.));
#2147=DIRECTION('center_axis',(0.,0.,-1.));
#2148=DIRECTION('ref_axis',(1.,0.,0.));
#2149=DIRECTION('center_axis',(0.,0.,1.));
#2150=DIRECTION('ref_axis',(1.,0.,0.));
#2151=DIRECTION('center_axis',(0.,0.,1.));
#2152=DIRECTION('ref_axis',(1.,0.,0.));
#2153=DIRECTION('',(0.,0.,1.));
#2154=DIRECTION('center_axis',(0.,0.,-1.));
#2155=DIRECTION('ref_axis',(1.,0.,0.));
#2156=DIRECTION('center_axis',(0.,0.,1.));
#2157=DIRECTION('ref_axis',(1.,0.,0.));
#2158=DIRECTION('center_axis',(0.,0.,1.));
#2159=DIRECTION('ref_axis',(1.,0.,0.));
#2160=DIRECTION('',(0.,0.,1.));
#2161=DIRECTION('center_axis',(0.,0.,-1.));
#2162=DIRECTION('ref_axis',(1.,0.,0.));
#2163=DIRECTION('center_axis',(0.,0.,1.));
#2164=DIRECTION('ref_axis',(1.,0.,0.));
#2165=DIRECTION('center_axis',(0.,0.,1.));
#2166=DIRECTION('ref_axis',(1.,0.,0.));
#2167=DIRECTION('',(0.,0.,1.));
#2168=DIRECTION('center_axis',(0.,0.,-1.));
#2169=DIRECTION('ref_axis',(1.,0.,0.));
#2170=DIRECTION('center_axis',(0.,0.,1.));
#2171=DIRECTION('ref_axis',(1.,0.,0.));
#2172=DIRECTION('center_axis',(0.,0.,1.));
#2173=DIRECTION('ref_axis',(1.,0.,0.));
#2174=DIRECTION('',(0.,0.,1.));
#2175=DIRECTION('center_axis',(0.,0.,-1.));
#2176=DIRECTION('ref_axis',(1.,0.,0.));
#2177=DIRECTION('center_axis',(0.,0.,1.));
#2178=DIRECTION('ref_axis',(1.,0.,0.));
#2179=DIRECTION('center_axis',(0.,0.,1.));
#2180=DIRECTION('ref_axis',(1.,0.,0.));
#2181=DIRECTION('',(0.,0.,1.));
#2182=DIRECTION('center_axis',(0.,0.,-1.));
#2183=DIRECTION('ref_axis',(1.,0.,0.));
#2184=DIRECTION('center_axis',(0.,0.,1.));
#2185=DIRECTION('ref_axis',(1.,0.,0.));
#2186=DIRECTION('center_axis',(0.,0.,1.));
#2187=DIRECTION('ref_axis',(1.,0.,0.));
#2188=DIRECTION('',(0.,0.,1.));
#2189=DIRECTION('center_axis',(0.,0.,-1.));
#2190=DIRECTION('ref_axis',(1.,0.,0.));
#2191=DIRECTION('center_axis',(0.,0.,1.));
#2192=DIRECTION('ref_axis',(1.,0.,0.));
#2193=DIRECTION('center_axis',(0.,0.,1.));
#2194=DIRECTION('ref_axis',(1.,0.,0.));
#2195=DIRECTION('',(0.,0.,1.));
#2196=DIRECTION('center_axis',(0.,0.,-1.));
#2197=DIRECTION('ref_axis',(1.,0.,0.));
#2198=DIRECTION('center_axis',(0.,1.,0.));
#2199=DIRECTION('ref_axis',(-1.,0.,0.));
#2200=DIRECTION('',(-1.,0.,0.));
#2201=DIRECTION('',(0.,0.,1.));
#2202=DIRECTION('',(-1.,0.,0.));
#2203=DIRECTION('',(0.,0.,1.));
#2204=DIRECTION('center_axis',(1.,0.,0.));
#2205=DIRECTION('ref_axis',(0.,1.,0.));
#2206=DIRECTION('',(0.,1.,0.));
#2207=DIRECTION('',(0.,1.,0.));
#2208=DIRECTION('',(0.,0.,1.));
#2209=DIRECTION('center_axis',(0.,-1.,0.));
#2210=DIRECTION('ref_axis',(1.,0.,0.));
#2211=DIRECTION('',(1.,0.,0.));
#2212=DIRECTION('',(1.,0.,0.));
#2213=DIRECTION('',(0.,0.,1.));
#2214=DIRECTION('center_axis',(-1.,0.,0.));
#2215=DIRECTION('ref_axis',(0.,-1.,0.));
#2216=DIRECTION('',(0.,-1.,0.));
#2217=DIRECTION('',(0.,-1.,0.));
#2218=DIRECTION('center_axis',(0.,0.,1.));
#2219=DIRECTION('ref_axis',(1.,0.,0.));
#2220=DIRECTION('center_axis',(0.,0.,1.));
#2221=DIRECTION('ref_axis',(1.,0.,0.));
#2503=CARTESIAN_POINT('',(0.,0.,0.));
#2504=CARTESIAN_POINT('Origin',(2.5,-1.5,-0.1));
#2505=CARTESIAN_POINT('',(2.225,-1.5,0.));
#2506=CARTESIAN_POINT('Origin',(2.5,-1.5,0.));
#2507=CARTESIAN_POINT('',(2.225,-1.5,1.));
#2508=CARTESIAN_POINT('',(2.225,-1.5,-0.1));
#2509=CARTESIAN_POINT('Origin',(2.5,-1.5,1.));
#2510=CARTESIAN_POINT('Origin',(0.5,1.5,-0.1));
#2511=CARTESIAN_POINT('',(0.225,1.5,0.));
#2512=CARTESIAN_POINT('Origin',(0.5,1.5,0.));
#2513=CARTESIAN_POINT('',(0.225,1.5,1.));
#2514=CARTESIAN_POINT('',(0.225,1.5,-0.1));
#2515=CARTESIAN_POINT('Origin',(0.5,1.5,1.));
#2516=CARTESIAN_POINT('Origin',(0.5,-1.5,-0.1));
#2517=CARTESIAN_POINT('',(0.225,-1.5,0.));
#2518=CARTESIAN_POINT('Origin',(0.5,-1.5,0.));
#2519=CARTESIAN_POINT('',(0.225,-1.5,1.));
#2520=CARTESIAN_POINT('',(0.225,-1.5,-0.1));
#2521=CARTESIAN_POINT('Origin',(0.5,-1.5,1.));
#2522=CARTESIAN_POINT('Origin',(2.5,1.5,-0.1));
#2523=CARTESIAN_POINT('',(2.225,1.5,0.));
#2524=CARTESIAN_POINT('Origin',(2.5,1.5,0.));
#2525=CARTESIAN_POINT('',(2.225,1.5,1.));
#2526=CARTESIAN_POINT('',(2.225,1.5,-0.1));
#2527=CARTESIAN_POINT('Origin',(2.5,1.5,1.));
#2528=CARTESIAN_POINT('Origin',(1.5,0.,-0.1));
#2529=CARTESIAN_POINT('',(1.16,-4.163799117101E-17,0.));
#2530=CARTESIAN_POINT('Origin',(1.5,0.,0.));
#2531=CARTESIAN_POINT('',(1.16,4.163799117101E-17,1.));
#2532=CARTESIAN_POINT('',(1.16,-4.163799117101E-17,-0.1));
#2533=CARTESIAN_POINT('Origin',(1.5,0.,1.));
#2534=CARTESIAN_POINT('Origin',(5.,2.5,-0.1));
#2535=CARTESIAN_POINT('',(4.66,2.5,0.));
#2536=CARTESIAN_POINT('Origin',(5.,2.5,0.));
#2537=CARTESIAN_POINT('',(4.66,2.5,1.));
#2538=CARTESIAN_POINT('',(4.66,2.5,-0.1));
#2539=CARTESIAN_POINT('Origin',(5.,2.5,1.));
#2540=CARTESIAN_POINT('Origin',(5.,-2.5,-0.1));
#2541=CARTESIAN_POINT('',(4.66,-2.5,0.));
#2542=CARTESIAN_POINT('Origin',(5.,-2.5,0.));
#2543=CARTESIAN_POINT('',(4.66,-2.5,1.));
#2544=CARTESIAN_POINT('',(4.66,-2.5,-0.1));
#2545=CARTESIAN_POINT('Origin',(5.,-2.5,1.));
#2546=CARTESIAN_POINT('Origin',(2.5,5.,-0.1));
#2547=CARTESIAN_POINT('',(2.16,5.,0.));
#2548=CARTESIAN_POINT('Origin',(2.5,5.,0.));
#2549=CARTESIAN_POINT('',(2.16,5.,1.));
#2550=CARTESIAN_POINT('',(2.16,5.,-0.1));
#2551=CARTESIAN_POINT('Origin',(2.5,5.,1.));
#2552=CARTESIAN_POINT('Origin',(2.5,0.,-0.1));
#2553=CARTESIAN_POINT('',(2.16,-4.163799117101E-17,0.));
#2554=CARTESIAN_POINT('Origin',(2.5,0.,0.));
#2555=CARTESIAN_POINT('',(2.16,4.163799117101E-17,1.));
#2556=CARTESIAN_POINT('',(2.16,-4.163799117101E-17,-0.1));
#2557=CARTESIAN_POINT('Origin',(2.5,0.,1.));
#2558=CARTESIAN_POINT('Origin',(2.5,-5.,-0.1));
#2559=CARTESIAN_POINT('',(2.16,-5.,0.));
#2560=CARTESIAN_POINT('Origin',(2.5,-5.,0.));
#2561=CARTESIAN_POINT('',(2.16,-5.,1.));
#2562=CARTESIAN_POINT('',(2.16,-5.,-0.1));
#2563=CARTESIAN_POINT('Origin',(2.5,-5.,1.));
#2564=CARTESIAN_POINT('Origin',(0.,2.5,-0.1));
#2565=CARTESIAN_POINT('',(-0.34,2.5,0.));
#2566=CARTESIAN_POINT('Origin',(0.,2.5,0.));
#2567=CARTESIAN_POINT('',(-0.34,2.5,1.));
#2568=CARTESIAN_POINT('',(-0.34,2.5,-0.1));
#2569=CARTESIAN_POINT('Origin',(0.,2.5,1.));
#2570=CARTESIAN_POINT('Origin',(0.,0.,-0.1));
#2571=CARTESIAN_POINT('',(-0.34,-4.163799117101E-17,0.));
#2572=CARTESIAN_POINT('Origin',(0.,0.,0.));
#2573=CARTESIAN_POINT('',(-0.34,4.163799117101E-17,1.));
#2574=CARTESIAN_POINT('',(-0.34,-4.163799117101E-17,-0.1));
#2575=CARTESIAN_POINT('Origin',(0.,0.,1.));
#2576=CARTESIAN_POINT('Origin',(0.,-5.,-0.1));
#2577=CARTESIAN_POINT('',(-0.34,-5.,0.));
#2578=CARTESIAN_POINT('Origin',(0.,-5.,0.));
#2579=CARTESIAN_POINT('',(-0.34,-5.,1.));
#2580=CARTESIAN_POINT('',(-0.34,-5.,-0.1));
#2581=CARTESIAN_POINT('Origin',(0.,-5.,1.));
#2582=CARTESIAN_POINT('Origin',(-2.5,2.5,-0.1));
#2583=CARTESIAN_POINT('',(-2.84,2.5,0.));
#2584=CARTESIAN_POINT('Origin',(-2.5,2.5,0.));
#2585=CARTESIAN_POINT('',(-2.84,2.5,1.));
#2586=CARTESIAN_POINT('',(-2.84,2.5,-0.1));
#2587=CARTESIAN_POINT('Origin',(-2.5,2.5,1.));
#2588=CARTESIAN_POINT('Origin',(-2.5,-2.5,-0.1));
#2589=CARTESIAN_POINT('',(-2.84,-2.5,0.));
#2590=CARTESIAN_POINT('Origin',(-2.5,-2.5,0.));
#2591=CARTESIAN_POINT('',(-2.84,-2.5,1.));
#2592=CARTESIAN_POINT('',(-2.84,-2.5,-0.1));
#2593=CARTESIAN_POINT('Origin',(-2.5,-2.5,1.));
#2594=CARTESIAN_POINT('Origin',(-5.,5.,-0.1));
#2595=CARTESIAN_POINT('',(-5.34,5.,0.));
#2596=CARTESIAN_POINT('Origin',(-5.,5.,0.));
#2597=CARTESIAN_POINT('',(-5.34,5.,1.));
#2598=CARTESIAN_POINT('',(-5.34,5.,-0.1));
#2599=CARTESIAN_POINT('Origin',(-5.,5.,1.));
#2600=CARTESIAN_POINT('Origin',(-5.,0.,-0.1));
#2601=CARTESIAN_POINT('',(-5.34,-4.163799117101E-17,0.));
#2602=CARTESIAN_POINT('Origin',(-5.,0.,0.));
#2603=CARTESIAN_POINT('',(-5.34,4.163799117101E-17,1.));
#2604=CARTESIAN_POINT('',(-5.34,-4.163799117101E-17,-0.1));
#2605=CARTESIAN_POINT('Origin',(-5.,0.,1.));
#2606=CARTESIAN_POINT('Origin',(-5.,-2.5,-0.1));
#2607=CARTESIAN_POINT('',(-5.34,-2.5,0.));
#2608=CARTESIAN_POINT('Origin',(-5.,-2.5,0.));
#2609=CARTESIAN_POINT('',(-5.34,-2.5,1.));
#2610=CARTESIAN_POINT('',(-5.34,-2.5,-0.1));
#2611=CARTESIAN_POINT('Origin',(-5.,-2.5,1.));
#2612=CARTESIAN_POINT('Origin',(-5.,2.5,-0.1));
#2613=CARTESIAN_POINT('',(-5.34,2.5,0.));
#2614=CARTESIAN_POINT('Origin',(-5.,2.5,0.));
#2615=CARTESIAN_POINT('',(-5.34,2.5,1.));
#2616=CARTESIAN_POINT('',(-5.34,2.5,-0.1));
#2617=CARTESIAN_POINT('Origin',(-5.,2.5,1.));
#2618=CARTESIAN_POINT('Origin',(-2.5,-5.,-0.1));
#2619=CARTESIAN_POINT('',(-2.84,-5.,0.));
#2620=CARTESIAN_POINT('Origin',(-2.5,-5.,0.));
#2621=CARTESIAN_POINT('',(-2.84,-5.,1.));
#2622=CARTESIAN_POINT('',(-2.84,-5.,-0.1));
#2623=CARTESIAN_POINT('Origin',(-2.5,-5.,1.));
#2624=CARTESIAN_POINT('Origin',(-2.5,0.,-0.1));
#2625=CARTESIAN_POINT('',(-2.84,-4.163799117101E-17,0.));
#2626=CARTESIAN_POINT('Origin',(-2.5,0.,0.));
#2627=CARTESIAN_POINT('',(-2.84,4.163799117101E-17,1.));
#2628=CARTESIAN_POINT('',(-2.84,-4.163799117101E-17,-0.1));
#2629=CARTESIAN_POINT('Origin',(-2.5,0.,1.));
#2630=CARTESIAN_POINT('Origin',(-2.5,5.,-0.1));
#2631=CARTESIAN_POINT('',(-2.84,5.,0.));
#2632=CARTESIAN_POINT('Origin',(-2.5,5.,0.));
#2633=CARTESIAN_POINT('',(-2.84,5.,1.));
#2634=CARTESIAN_POINT('',(-2.84,5.,-0.1));
#2635=CARTESIAN_POINT('Origin',(-2.5,5.,1.));
#2636=CARTESIAN_POINT('Origin',(0.,-2.5,-0.1));
#2637=CARTESIAN_POINT('',(-0.34,-2.5,0.));
#2638=CARTESIAN_POINT('Origin',(0.,-2.5,0.));
#2639=CARTESIAN_POINT('',(-0.34,-2.5,1.));
#2640=CARTESIAN_POINT('',(-0.34,-2.5,-0.1));
#2641=CARTESIAN_POINT('Origin',(0.,-2.5,1.));
#2642=CARTESIAN_POINT('Origin',(-5.,-5.,-0.1));
#2643=CARTESIAN_POINT('',(-5.34,-5.,0.));
#2644=CARTESIAN_POINT('Origin',(-5.,-5.,0.));
#2645=CARTESIAN_POINT('',(-5.34,-5.,1.));
#2646=CARTESIAN_POINT('',(-5.34,-5.,-0.1));
#2647=CARTESIAN_POINT('Origin',(-5.,-5.,1.));
#2648=CARTESIAN_POINT('Origin',(0.,5.,-0.1));
#2649=CARTESIAN_POINT('',(-0.34,5.,0.));
#2650=CARTESIAN_POINT('Origin',(0.,5.,0.));
#2651=CARTESIAN_POINT('',(-0.34,5.,1.));
#2652=CARTESIAN_POINT('',(-0.34,5.,-0.1));
#2653=CARTESIAN_POINT('Origin',(0.,5.,1.));
#2654=CARTESIAN_POINT('Origin',(2.5,-2.5,-0.1));
#2655=CARTESIAN_POINT('',(2.16,-2.5,0.));
#2656=CARTESIAN_POINT('Origin',(2.5,-2.5,0.));
#2657=CARTESIAN_POINT('',(2.16,-2.5,1.));
#2658=CARTESIAN_POINT('',(2.16,-2.5,-0.1));
#2659=CARTESIAN_POINT('Origin',(2.5,-2.5,1.));
#2660=CARTESIAN_POINT('Origin',(2.5,2.5,-0.1));
#2661=CARTESIAN_POINT('',(2.16,2.5,0.));
#2662=CARTESIAN_POINT('Origin',(2.5,2.5,0.));
#2663=CARTESIAN_POINT('',(2.16,2.5,1.));
#2664=CARTESIAN_POINT('',(2.16,2.5,-0.1));
#2665=CARTESIAN_POINT('Origin',(2.5,2.5,1.));
#2666=CARTESIAN_POINT('Origin',(5.,-5.,-0.1));
#2667=CARTESIAN_POINT('',(4.66,-5.,0.));
#2668=CARTESIAN_POINT('Origin',(5.,-5.,0.));
#2669=CARTESIAN_POINT('',(4.66,-5.,1.));
#2670=CARTESIAN_POINT('',(4.66,-5.,-0.1));
#2671=CARTESIAN_POINT('Origin',(5.,-5.,1.));
#2672=CARTESIAN_POINT('Origin',(5.,0.,-0.1));
#2673=CARTESIAN_POINT('',(4.66,-4.163799117101E-17,0.));
#2674=CARTESIAN_POINT('Origin',(5.,0.,0.));
#2675=CARTESIAN_POINT('',(4.66,4.163799117101E-17,1.));
#2676=CARTESIAN_POINT('',(4.66,-4.163799117101E-17,-0.1));
#2677=CARTESIAN_POINT('Origin',(5.,0.,1.));
#2678=CARTESIAN_POINT('Origin',(5.,5.,-0.1));
#2679=CARTESIAN_POINT('',(4.66,5.,0.));
#2680=CARTESIAN_POINT('Origin',(5.,5.,0.));
#2681=CARTESIAN_POINT('',(4.66,5.,1.));
#2682=CARTESIAN_POINT('',(4.66,5.,-0.1));
#2683=CARTESIAN_POINT('Origin',(5.,5.,1.));
#2684=CARTESIAN_POINT('Origin',(7.5,7.5,0.));
#2685=CARTESIAN_POINT('',(7.5,7.5,0.));
#2686=CARTESIAN_POINT('',(-7.5,7.5,0.));
#2687=CARTESIAN_POINT('',(7.5,7.5,0.));
#2688=CARTESIAN_POINT('',(-7.5,7.5,1.));
#2689=CARTESIAN_POINT('',(-7.5,7.5,0.));
#2690=CARTESIAN_POINT('',(7.5,7.5,1.));
#2691=CARTESIAN_POINT('',(7.5,7.5,1.));
#2692=CARTESIAN_POINT('',(7.5,7.5,0.));
#2693=CARTESIAN_POINT('Origin',(7.5,-7.5,0.));
#2694=CARTESIAN_POINT('',(7.5,-7.5,0.));
#2695=CARTESIAN_POINT('',(7.5,-7.5,0.));
#2696=CARTESIAN_POINT('',(7.5,-7.5,1.));
#2697=CARTESIAN_POINT('',(7.5,-7.5,1.));
#2698=CARTESIAN_POINT('',(7.5,-7.5,0.));
#2699=CARTESIAN_POINT('Origin',(-7.5,-7.5,0.));
#2700=CARTESIAN_POINT('',(-7.5,-7.5,0.));
#2701=CARTESIAN_POINT('',(-7.5,-7.5,0.));
#2702=CARTESIAN_POINT('',(-7.5,-7.5,1.));
#2703=CARTESIAN_POINT('',(-7.5,-7.5,1.));
#2704=CARTESIAN_POINT('',(-7.5,-7.5,0.));
#2705=CARTESIAN_POINT('Origin',(-7.5,7.5,0.));
#2706=CARTESIAN_POINT('',(-7.5,7.5,0.));
#2707=CARTESIAN_POINT('',(-7.5,7.5,1.));
#2708=CARTESIAN_POINT('Origin',(0.,0.,1.));
#2709=CARTESIAN_POINT('Origin',(0.,0.,0.));
#2981=UNCERTAINTY_MEASURE_WITH_UNIT(LENGTH_MEASURE(0.001),#2997,
'DISTANCE_ACCURACY_VALUE',
'Maximum model space distance between geometric entities at asserted c
onnectivities');
#2987=UNCERTAINTY_MEASURE_WITH_UNIT(LENGTH_MEASURE(0.001),#2997,
'DISTANCE_ACCURACY_VALUE',
'Maximum model space distance between geometric entities at asserted c
onnectivities');
#2990=(
GEOMETRIC_REPRESENTATION_CONTEXT(3)
GLOBAL_UNCERTAINTY_ASSIGNED_CONTEXT((#2981))
GLOBAL_UNIT_ASSIGNED_CONTEXT((#2997,#2999,#3000))
REPRESENTATION_CONTEXT('','3D')
);
#2996=(
GEOMETRIC_REPRESENTATION_CONTEXT(3)
GLOBAL_UNCERTAINTY_ASSIGNED_CONTEXT((#2987))
GLOBAL_UNIT_ASSIGNED_CONTEXT((#2997,#2999,#3000))
REPRESENTATION_CONTEXT('','3D')
);
#2997=(
LENGTH_UNIT()
NAMED_UNIT(*)
SI_UNIT(.CENTI.,.METRE.)
);
#2999=(
NAMED_UNIT(*)
PLANE_ANGLE_UNIT()
SI_UNIT($,.RADIAN.)
);
#3000=(
NAMED_UNIT(*)
SI_UNIT($,.STERADIAN.)
SOLID_ANGLE_UNIT()
);
#3003=SHAPE_DEFINITION_REPRESENTATION(#3011,#3029);
#3011=PRODUCT_DEFINITION_SHAPE('',$,#3038);
#3029=SHAPE_REPRESENTATION('',(#1784),#2990);
#3035=PRODUCT_DEFINITION_CONTEXT('part definition',#3061,'design');
#3038=PRODUCT_DEFINITION('Fixture grid plate','Fixture grid plate',#3046,
#3035);
#3046=PRODUCT_DEFINITION_FORMATION('',$,#3065);
#3061=APPLICATION_CONTEXT(
'Core Data for Automotive Mechanical Design Process');
#3062=PRODUCT_CONTEXT('part definition',#3061,'mechanical');
#3065=PRODUCT('Fixture grid plate','Fixture grid plate',
'Fixture grid plate',(#3062));
#3134=COLOUR_RGB('Off White',0.89,0.88,0.83);
#3135=FILL_AREA_STYLE_COLOUR('',#3134);
#3136=FILL_AREA_STYLE('',(#3135));
#3137=SURFACE_STYLE_FILL_AREA(#3136);
#3138=SURFACE_SIDE_STYLE('',(#3137));
#3139=SURFACE_STYLE_USAGE(.BOTH.,#3138);
#3140=PRESENTATION_STYLE_ASSIGNMENT((#3139));
ENDSEC;
END-ISO-10303-21;
